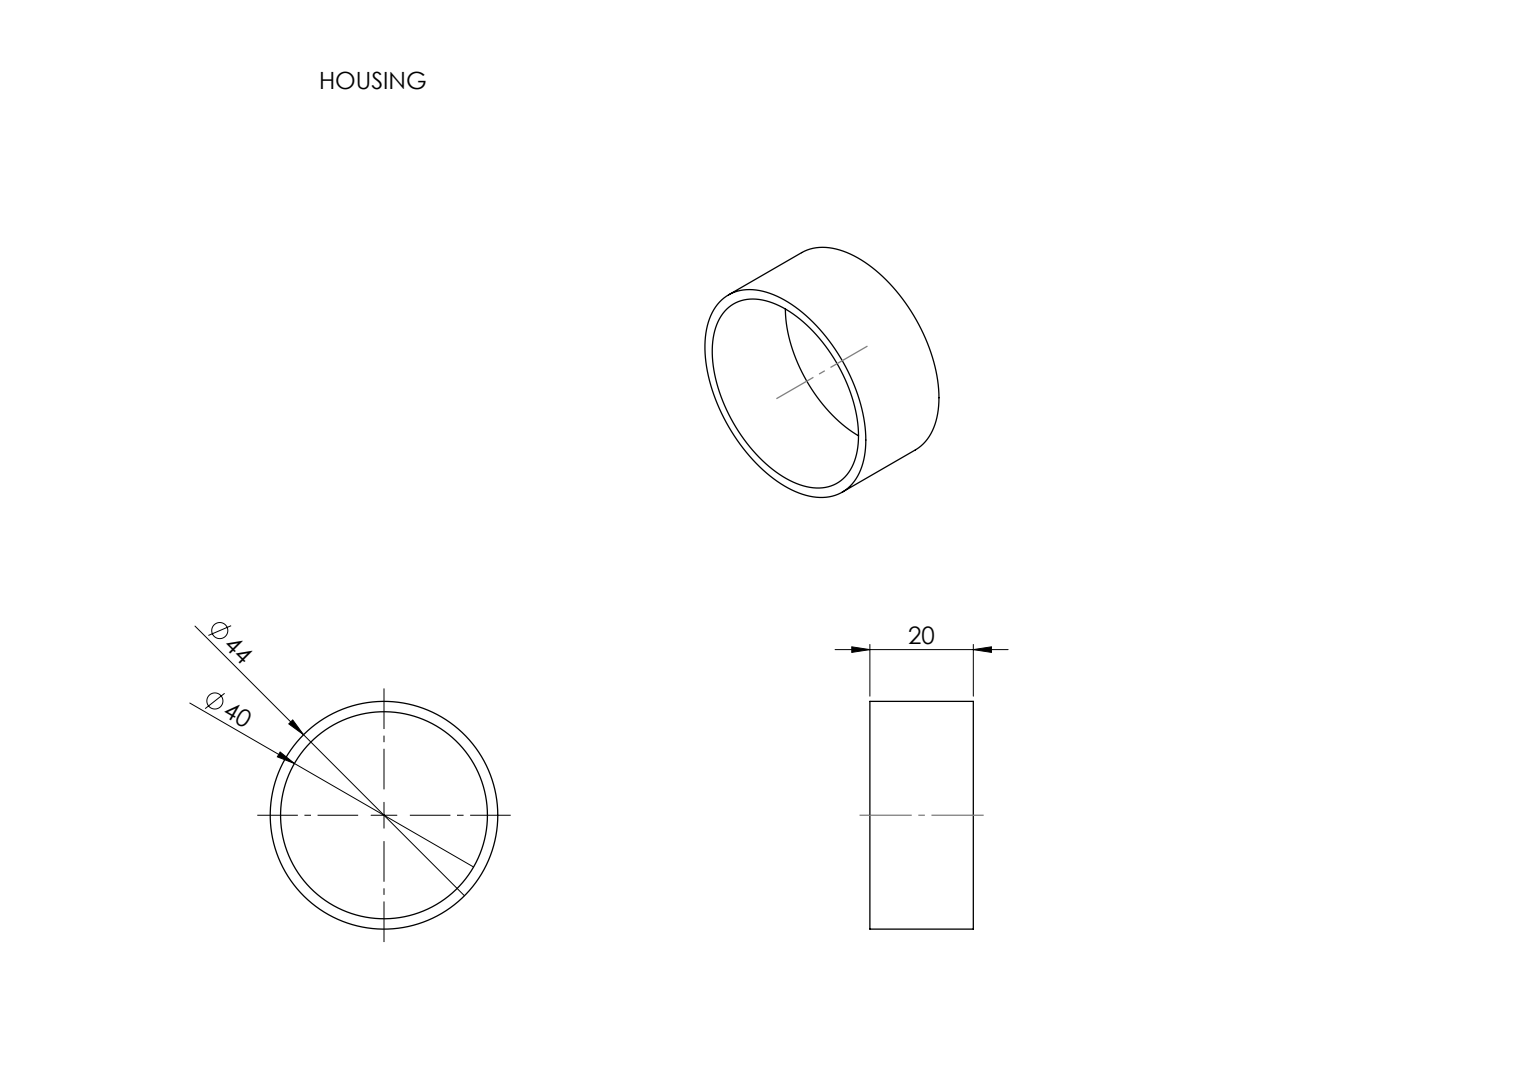
ISO-10303-21;
HEADER;
FILE_DESCRIPTION (('STEP AP214'),
    '1' );
FILE_NAME ('housing.step',
    '2026-10-08T12:30:53',
    ( '' ),
    ( '' ),
    'SwSTEP 2.0',
    'SolidWorks 2026',
    '' );
FILE_SCHEMA (( 'AUTOMOTIVE_DESIGN' ));
ENDSEC;

DATA;
#96=ORIENTED_EDGE ( 'NONE', *, *, #6796, .F. ) ;
#313=CARTESIAN_POINT ( 'NONE',  ( 0.000000000000000000, 0.000000000000000000, 20.00000000000000000 ) ) ;
#321=CARTESIAN_POINT ( 'NONE',  ( 0.000000000000000000, 0.000000000000000000, 20.00000000000000000 ) ) ;
#331=CARTESIAN_POINT ( 'NONE',  ( 0.000000000000000000, 0.000000000000000000, 20.00000000000000000 ) ) ;
#339=AXIS2_PLACEMENT_3D ( 'NONE', #331, #5047, #8783 ) ;
#478=UNCERTAINTY_MEASURE_WITH_UNIT (LENGTH_MEASURE( 1.000000000000000082E-05 ), #5286, 'distance_accuracy_value', 'NONE');
#542=DIRECTION ( 'NONE',  ( 1.000000000000000000, 0.000000000000000000, 0.000000000000000000 ) ) ;
#621=FILL_AREA_STYLE ('',( #9865 ) ) ;
#694=SURFACE_STYLE_USAGE ( .BOTH. , #4367 ) ;
#720=PRODUCT_DEFINITION_CONTEXT ( 'detailed design', #10992, 'design' ) ;
#831=CARTESIAN_POINT ( 'NONE',  ( 19.99999999999999645, 2.449293598294706119E-15, 20.00000000000000000 ) ) ;
#894=FACE_OUTER_BOUND ( 'NONE', #9272, .T. ) ;
#945=DIRECTION ( 'NONE',  ( -0.000000000000000000, -0.000000000000000000, -1.000000000000000000 ) ) ;
#949=EDGE_LOOP ( 'NONE', ( #11530, #8082, #9226, #7103 ) ) ;
#993=CIRCLE ( 'NONE', #10561, 19.99999999999999645 ) ;
#1170=VERTEX_POINT ( 'NONE', #5918 ) ;
#1179=AXIS2_PLACEMENT_3D ( 'NONE', #3701, #8417, #7546 ) ;
#1190=PLANE ( 'NONE',  #7958 ) ;
#1294=CIRCLE ( 'NONE', #7739, 19.99999999999999645 ) ;
#1477=PRESENTATION_STYLE_ASSIGNMENT (( #10268 ) ) ;
#1490=( NAMED_UNIT ( * ) SI_UNIT ( $, .STERADIAN. ) SOLID_ANGLE_UNIT ( ) );
#1492=EDGE_CURVE ( 'NONE', #10594, #10386, #9022, .T. ) ;
#1514=PRODUCT_CONTEXT ( 'NONE', #2788, 'mechanical' ) ;
#1548=MECHANICAL_DESIGN_GEOMETRIC_PRESENTATION_REPRESENTATION('',(#9368),#5064);
#1551=DIRECTION ( 'NONE',  ( 0.000000000000000000, 0.000000000000000000, 1.000000000000000000 ) ) ;
#1565=ADVANCED_FACE ( 'NONE', ( #7489 ), #10304, .F. ) ;
#1574=EDGE_CURVE ( 'NONE', #8389, #10578, #8998, .T. ) ;
#1616=AXIS2_PLACEMENT_3D ( 'NONE', #2628, #6184, #542 ) ;
#1674=CARTESIAN_POINT ( 'NONE',  ( 0.000000000000000000, 0.000000000000000000, 0.000000000000000000 ) ) ;
#1759=ADVANCED_FACE ( 'NONE', ( #5901 ), #4004, .F. ) ;
#1811=( GEOMETRIC_REPRESENTATION_CONTEXT ( 3 ) GLOBAL_UNCERTAINTY_ASSIGNED_CONTEXT ( ( #478 ) ) GLOBAL_UNIT_ASSIGNED_CONTEXT ( ( #5286, #9878, #2599 ) ) REPRESENTATION_CONTEXT ( 'NONE', 'WORKASPACE' ) );
#1812=FACE_BOUND ( 'NONE', #10883, .T. ) ;
#1825=( NAMED_UNIT ( * ) PLANE_ANGLE_UNIT ( ) SI_UNIT ( $, .RADIAN. ) );
#1826=UNCERTAINTY_MEASURE_WITH_UNIT (LENGTH_MEASURE( 1.000000000000000082E-05 ), #3721, 'distance_accuracy_value', 'NONE');
#1955=ORIENTED_EDGE ( 'NONE', *, *, #1574, .T. ) ;
#2025=EDGE_CURVE ( 'NONE', #6334, #10386, #3812, .T. ) ;
#2134=CARTESIAN_POINT ( 'NONE',  ( 0.000000000000000000, 0.000000000000000000, 20.00000000000000000 ) ) ;
#2153=DIRECTION ( 'NONE',  ( 1.000000000000000000, 0.000000000000000000, 0.000000000000000000 ) ) ;
#2166=VECTOR ( 'NONE', #10232, 1000.000000000000000 ) ;
#2182=FACE_OUTER_BOUND ( 'NONE', #5458, .T. ) ;
#2199=FACE_OUTER_BOUND ( 'NONE', #949, .T. ) ;
#2216=AXIS2_PLACEMENT_3D ( 'NONE', #2134, #10519, #10760 ) ;
#2332=VECTOR ( 'NONE', #7364, 1000.000000000000000 ) ;
#2396=EDGE_CURVE ( 'NONE', #10386, #10594, #993, .T. ) ;
#2505=CARTESIAN_POINT ( 'NONE',  ( 0.000000000000000000, 0.000000000000000000, 0.000000000000000000 ) ) ;
#2508=CARTESIAN_POINT ( 'NONE',  ( 19.99999999999999645, 2.449293598294706119E-15, 20.00000000000000000 ) ) ;
#2599=( NAMED_UNIT ( * ) SI_UNIT ( $, .STERADIAN. ) SOLID_ANGLE_UNIT ( ) );
#2628=CARTESIAN_POINT ( 'NONE',  ( 0.000000000000000000, 0.000000000000000000, 20.00000000000000000 ) ) ;
#2653=DIRECTION ( 'NONE',  ( 1.000000000000000000, 0.000000000000000000, 0.000000000000000000 ) ) ;
#2679=SURFACE_SIDE_STYLE ('',( #5212 ) ) ;
#2709=VECTOR ( 'NONE', #7824, 1000.000000000000000 ) ;
#2743=AXIS2_PLACEMENT_3D ( 'NONE', #8356, #945, #3767 ) ;
#2788=APPLICATION_CONTEXT ( 'automotive_design' ) ;
#2839=FACE_OUTER_BOUND ( 'NONE', #6431, .T. ) ;
#2852=CARTESIAN_POINT ( 'NONE',  ( 0.000000000000000000, 0.000000000000000000, 20.00000000000000000 ) ) ;
#2998=ORIENTED_EDGE ( 'NONE', *, *, #1492, .T. ) ;
#3105=ORIENTED_EDGE ( 'NONE', *, *, #8115, .F. ) ;
#3124=CIRCLE ( 'NONE', #7411, 22.00000000000000000 ) ;
#3188=COLOUR_RGB ( '', 0.72549020, 0.75294118, 0.79215686) ;
#3482=EDGE_LOOP ( 'NONE', ( #7823, #9576, #6820, #10091 ) ) ;
#3495=DIRECTION ( 'NONE',  ( 0.000000000000000000, 0.000000000000000000, 1.000000000000000000 ) ) ;
#3497=ORIENTED_EDGE ( 'NONE', *, *, #9146, .F. ) ;
#3547=CIRCLE ( 'NONE', #6281, 19.99999999999999645 ) ;
#3615=ORIENTED_EDGE ( 'NONE', *, *, #5180, .F. ) ;
#3643=CARTESIAN_POINT ( 'NONE',  ( 0.000000000000000000, 0.000000000000000000, 0.000000000000000000 ) ) ;
#3672=ORIENTED_EDGE ( 'NONE', *, *, #1574, .F. ) ;
#3692=AXIS2_PLACEMENT_3D ( 'NONE', #6399, #5550, #3710 ) ;
#3701=CARTESIAN_POINT ( 'NONE',  ( 0.000000000000000000, 0.000000000000000000, 0.000000000000000000 ) ) ;
#3710=DIRECTION ( 'NONE',  ( 1.000000000000000000, 0.000000000000000000, -0.000000000000000000 ) ) ;
#3721=( LENGTH_UNIT ( ) NAMED_UNIT ( * ) SI_UNIT ( .MILLI., .METRE. ) );
#3724=CARTESIAN_POINT ( 'NONE',  ( 19.99999999999999645, 2.449293598294706119E-15, 0.000000000000000000 ) ) ;
#3767=DIRECTION ( 'NONE',  ( -1.000000000000000000, 0.000000000000000000, 0.000000000000000000 ) ) ;
#3812=LINE ( 'NONE', #5584, #2166 ) ;
#3830=EDGE_CURVE ( 'NONE', #6334, #3911, #3547, .T. ) ;
#3872=DIRECTION ( 'NONE',  ( -1.000000000000000000, 0.000000000000000000, 0.000000000000000000 ) ) ;
#3911=VERTEX_POINT ( 'NONE', #2508 ) ;
#4004=CYLINDRICAL_SURFACE ( 'NONE', #8423, 19.99999999999999645 ) ;
#4123=DIRECTION ( 'NONE',  ( -0.000000000000000000, -0.000000000000000000, -1.000000000000000000 ) ) ;
#4260=CARTESIAN_POINT ( 'NONE',  ( -22.00000000000000000, 0.000000000000000000, 20.00000000000000000 ) ) ;
#4367=SURFACE_SIDE_STYLE ('',( #11042 ) ) ;
#4427=SHAPE_REPRESENTATION_RELATIONSHIP ( 'NONE' , 'NONE' ,  #5127, #6320 ) ;
#4454=DIRECTION ( 'NONE',  ( 0.000000000000000000, 0.000000000000000000, 1.000000000000000000 ) ) ;
#4502=AXIS2_PLACEMENT_3D ( 'NONE', #3643, #12018, #6393 ) ;
#4529=CLOSED_SHELL ( 'NONE', ( #1759, #5007, #6067, #8839, #6656, #1565 ) ) ;
#4673=CARTESIAN_POINT ( 'NONE',  ( 0.000000000000000000, 0.000000000000000000, 20.00000000000000000 ) ) ;
#4752=DIRECTION ( 'NONE',  ( 0.000000000000000000, 0.000000000000000000, 1.000000000000000000 ) ) ;
#4980=LINE ( 'NONE', #8833, #6405 ) ;
#5007=ADVANCED_FACE ( 'NONE', ( #2199 ), #11673, .T. ) ;
#5047=DIRECTION ( 'NONE',  ( 0.000000000000000000, 0.000000000000000000, 1.000000000000000000 ) ) ;
#5064=( GEOMETRIC_REPRESENTATION_CONTEXT ( 3 ) GLOBAL_UNCERTAINTY_ASSIGNED_CONTEXT ( ( #1826 ) ) GLOBAL_UNIT_ASSIGNED_CONTEXT ( ( #3721, #1825, #5499 ) ) REPRESENTATION_CONTEXT ( 'NONE', 'WORKASPACE' ) );
#5127=SHAPE_REPRESENTATION ( 'housing', ( #8474 ), #5529 ) ;
#5180=EDGE_CURVE ( 'NONE', #10578, #8389, #3124, .T. ) ;
#5205=DIRECTION ( 'NONE',  ( 1.000000000000000000, 0.000000000000000000, 0.000000000000000000 ) ) ;
#5212=SURFACE_STYLE_FILL_AREA ( #621 ) ;
#5286=( LENGTH_UNIT ( ) NAMED_UNIT ( * ) SI_UNIT ( .MILLI., .METRE. ) );
#5381=DIRECTION ( 'NONE',  ( 1.000000000000000000, 0.000000000000000000, 0.000000000000000000 ) ) ;
#5382=UNCERTAINTY_MEASURE_WITH_UNIT (LENGTH_MEASURE( 1.000000000000000082E-05 ), #10980, 'distance_accuracy_value', 'NONE');
#5458=EDGE_LOOP ( 'NONE', ( #8805, #11887 ) ) ;
#5499=( NAMED_UNIT ( * ) SI_UNIT ( $, .STERADIAN. ) SOLID_ANGLE_UNIT ( ) );
#5529=( GEOMETRIC_REPRESENTATION_CONTEXT ( 3 ) GLOBAL_UNCERTAINTY_ASSIGNED_CONTEXT ( ( #5382 ) ) GLOBAL_UNIT_ASSIGNED_CONTEXT ( ( #10980, #10861, #1490 ) ) REPRESENTATION_CONTEXT ( 'NONE', 'WORKASPACE' ) );
#5550=DIRECTION ( 'NONE',  ( 0.000000000000000000, 0.000000000000000000, 1.000000000000000000 ) ) ;
#5584=CARTESIAN_POINT ( 'NONE',  ( -19.99999999999999645, 0.000000000000000000, 20.00000000000000000 ) ) ;
#5713=ORIENTED_EDGE ( 'NONE', *, *, #9658, .T. ) ;
#5901=FACE_OUTER_BOUND ( 'NONE', #8272, .T. ) ;
#5918=CARTESIAN_POINT ( 'NONE',  ( 22.00000000000000000, 2.694222958124176809E-15, 20.00000000000000000 ) ) ;
#5967=CARTESIAN_POINT ( 'NONE',  ( -19.99999999999999645, 0.000000000000000000, 20.00000000000000000 ) ) ;
#6067=ADVANCED_FACE ( 'NONE', ( #2182, #8546 ), #1190, .T. ) ;
#6110=STYLED_ITEM ( 'NONE', ( #8104 ), #6320 ) ;
#6116=CARTESIAN_POINT ( 'NONE',  ( -22.00000000000000000, 0.000000000000000000, 0.000000000000000000 ) ) ;
#6184=DIRECTION ( 'NONE',  ( 0.000000000000000000, 0.000000000000000000, 1.000000000000000000 ) ) ;
#6205=FILL_AREA_STYLE ('',( #7350 ) ) ;
#6243=COLOUR_RGB ( '', 0.72549020, 0.75294118, 0.79215686) ;
#6245=DIRECTION ( 'NONE',  ( 0.000000000000000000, 0.000000000000000000, 1.000000000000000000 ) ) ;
#6281=AXIS2_PLACEMENT_3D ( 'NONE', #7658, #3495, #5205 ) ;
#6320=ADVANCED_BREP_SHAPE_REPRESENTATION ( '', ( #8430, #8474 ), #5529 ) ;
#6334=VERTEX_POINT ( 'NONE', #5967 ) ;
#6393=DIRECTION ( 'NONE',  ( 1.000000000000000000, 0.000000000000000000, 0.000000000000000000 ) ) ;
#6399=CARTESIAN_POINT ( 'NONE',  ( 0.000000000000000000, 0.000000000000000000, 0.000000000000000000 ) ) ;
#6405=VECTOR ( 'NONE', #11638, 1000.000000000000000 ) ;
#6412=CARTESIAN_POINT ( 'NONE',  ( 0.000000000000000000, 0.000000000000000000, 0.000000000000000000 ) ) ;
#6431=EDGE_LOOP ( 'NONE', ( #3105, #3497, #5713, #1955 ) ) ;
#6617=ORIENTED_EDGE ( 'NONE', *, *, #2025, .F. ) ;
#6656=ADVANCED_FACE ( 'NONE', ( #2839 ), #8590, .T. ) ;
#6796=EDGE_CURVE ( 'NONE', #3911, #6334, #1294, .T. ) ;
#6820=ORIENTED_EDGE ( 'NONE', *, *, #2025, .T. ) ;
#6821=ORIENTED_EDGE ( 'NONE', *, *, #3830, .F. ) ;
#6880=CIRCLE ( 'NONE', #1616, 22.00000000000000000 ) ;
#6902=CARTESIAN_POINT ( 'NONE',  ( 22.00000000000000000, 2.694222958124176809E-15, 20.00000000000000000 ) ) ;
#7103=ORIENTED_EDGE ( 'NONE', *, *, #9658, .F. ) ;
#7244=PLANE ( 'NONE',  #3692 ) ;
#7350=FILL_AREA_STYLE_COLOUR ( '', #3188 ) ;
#7364=DIRECTION ( 'NONE',  ( -0.000000000000000000, -0.000000000000000000, -1.000000000000000000 ) ) ;
#7411=AXIS2_PLACEMENT_3D ( 'NONE', #6412, #4454, #5381 ) ;
#7475=MECHANICAL_DESIGN_GEOMETRIC_PRESENTATION_REPRESENTATION('',(#6110),#1811);
#7489=FACE_OUTER_BOUND ( 'NONE', #3482, .T. ) ;
#7546=DIRECTION ( 'NONE',  ( 1.000000000000000000, 0.000000000000000000, 0.000000000000000000 ) ) ;
#7658=CARTESIAN_POINT ( 'NONE',  ( 0.000000000000000000, 0.000000000000000000, 20.00000000000000000 ) ) ;
#7687=ORIENTED_EDGE ( 'NONE', *, *, #2396, .F. ) ;
#7739=AXIS2_PLACEMENT_3D ( 'NONE', #313, #10535, #2153 ) ;
#7764=ORIENTED_EDGE ( 'NONE', *, *, #8315, .T. ) ;
#7823=ORIENTED_EDGE ( 'NONE', *, *, #8315, .F. ) ;
#7824=DIRECTION ( 'NONE',  ( -0.000000000000000000, -0.000000000000000000, -1.000000000000000000 ) ) ;
#7842=VERTEX_POINT ( 'NONE', #4260 ) ;
#7958=AXIS2_PLACEMENT_3D ( 'NONE', #2852, #4752, #11351 ) ;
#8082=ORIENTED_EDGE ( 'NONE', *, *, #8115, .T. ) ;
#8104=PRESENTATION_STYLE_ASSIGNMENT (( #694 ) ) ;
#8115=EDGE_CURVE ( 'NONE', #1170, #10578, #9666, .T. ) ;
#8272=EDGE_LOOP ( 'NONE', ( #10399, #7764, #7687, #6617 ) ) ;
#8315=EDGE_CURVE ( 'NONE', #3911, #10594, #11798, .T. ) ;
#8356=CARTESIAN_POINT ( 'NONE',  ( 0.000000000000000000, 0.000000000000000000, 20.00000000000000000 ) ) ;
#8389=VERTEX_POINT ( 'NONE', #6116 ) ;
#8417=DIRECTION ( 'NONE',  ( 0.000000000000000000, 0.000000000000000000, 1.000000000000000000 ) ) ;
#8418=ORIENTED_EDGE ( 'NONE', *, *, #2396, .T. ) ;
#8423=AXIS2_PLACEMENT_3D ( 'NONE', #321, #4123, #11590 ) ;
#8430=MANIFOLD_SOLID_BREP ( 'Extrude-Thin1', #4529 ) ;
#8474=AXIS2_PLACEMENT_3D ( 'NONE', #1674, #1551, #2653 ) ;
#8531=DIRECTION ( 'NONE',  ( -0.000000000000000000, -0.000000000000000000, -1.000000000000000000 ) ) ;
#8546=FACE_BOUND ( 'NONE', #11852, .T. ) ;
#8590=CYLINDRICAL_SURFACE ( 'NONE', #10283, 22.00000000000000000 ) ;
#8783=DIRECTION ( 'NONE',  ( 1.000000000000000000, 0.000000000000000000, 0.000000000000000000 ) ) ;
#8805=ORIENTED_EDGE ( 'NONE', *, *, #9146, .T. ) ;
#8833=CARTESIAN_POINT ( 'NONE',  ( -22.00000000000000000, 0.000000000000000000, 20.00000000000000000 ) ) ;
#8839=ADVANCED_FACE ( 'NONE', ( #894, #1812 ), #7244, .F. ) ;
#8998=CIRCLE ( 'NONE', #1179, 22.00000000000000000 ) ;
#9022=CIRCLE ( 'NONE', #4502, 19.99999999999999645 ) ;
#9106=SHAPE_DEFINITION_REPRESENTATION ( #11470, #5127 ) ;
#9146=EDGE_CURVE ( 'NONE', #7842, #1170, #10702, .T. ) ;
#9189=PRODUCT_DEFINITION_FORMATION_WITH_SPECIFIED_SOURCE ( 'ANY', '', #9411, .NOT_KNOWN. ) ;
#9226=ORIENTED_EDGE ( 'NONE', *, *, #5180, .T. ) ;
#9272=EDGE_LOOP ( 'NONE', ( #3672, #3615 ) ) ;
#9368=STYLED_ITEM ( 'NONE', ( #1477 ), #8430 ) ;
#9411=PRODUCT ( 'housing', 'housing', '', ( #1514 ) ) ;
#9576=ORIENTED_EDGE ( 'NONE', *, *, #6796, .T. ) ;
#9658=EDGE_CURVE ( 'NONE', #7842, #8389, #4980, .T. ) ;
#9666=LINE ( 'NONE', #6902, #2709 ) ;
#9865=FILL_AREA_STYLE_COLOUR ( '', #6243 ) ;
#9878=( NAMED_UNIT ( * ) PLANE_ANGLE_UNIT ( ) SI_UNIT ( $, .RADIAN. ) );
#10082=CARTESIAN_POINT ( 'NONE',  ( -19.99999999999999645, 0.000000000000000000, 0.000000000000000000 ) ) ;
#10091=ORIENTED_EDGE ( 'NONE', *, *, #1492, .F. ) ;
#10232=DIRECTION ( 'NONE',  ( -0.000000000000000000, -0.000000000000000000, -1.000000000000000000 ) ) ;
#10268=SURFACE_STYLE_USAGE ( .BOTH. , #2679 ) ;
#10283=AXIS2_PLACEMENT_3D ( 'NONE', #4673, #8531, #3872 ) ;
#10304=CYLINDRICAL_SURFACE ( 'NONE', #2743, 19.99999999999999645 ) ;
#10317=PRODUCT_DEFINITION ( 'UNKNOWN', '', #9189, #720 ) ;
#10386=VERTEX_POINT ( 'NONE', #10082 ) ;
#10399=ORIENTED_EDGE ( 'NONE', *, *, #3830, .T. ) ;
#10519=DIRECTION ( 'NONE',  ( -0.000000000000000000, -0.000000000000000000, -1.000000000000000000 ) ) ;
#10535=DIRECTION ( 'NONE',  ( 0.000000000000000000, 0.000000000000000000, 1.000000000000000000 ) ) ;
#10561=AXIS2_PLACEMENT_3D ( 'NONE', #2505, #6245, #12104 ) ;
#10578=VERTEX_POINT ( 'NONE', #11312 ) ;
#10594=VERTEX_POINT ( 'NONE', #3724 ) ;
#10702=CIRCLE ( 'NONE', #339, 22.00000000000000000 ) ;
#10760=DIRECTION ( 'NONE',  ( -1.000000000000000000, 0.000000000000000000, 0.000000000000000000 ) ) ;
#10861=( NAMED_UNIT ( * ) PLANE_ANGLE_UNIT ( ) SI_UNIT ( $, .RADIAN. ) );
#10883=EDGE_LOOP ( 'NONE', ( #8418, #2998 ) ) ;
#10980=( LENGTH_UNIT ( ) NAMED_UNIT ( * ) SI_UNIT ( .MILLI., .METRE. ) );
#10992=APPLICATION_CONTEXT ( 'automotive_design' ) ;
#11042=SURFACE_STYLE_FILL_AREA ( #6205 ) ;
#11312=CARTESIAN_POINT ( 'NONE',  ( 22.00000000000000000, 2.694222958124176809E-15, 0.000000000000000000 ) ) ;
#11351=DIRECTION ( 'NONE',  ( 1.000000000000000000, 0.000000000000000000, -0.000000000000000000 ) ) ;
#11470=PRODUCT_DEFINITION_SHAPE ( 'NONE', 'NONE',  #10317 ) ;
#11530=ORIENTED_EDGE ( 'NONE', *, *, #11840, .F. ) ;
#11590=DIRECTION ( 'NONE',  ( -1.000000000000000000, 0.000000000000000000, 0.000000000000000000 ) ) ;
#11638=DIRECTION ( 'NONE',  ( -0.000000000000000000, -0.000000000000000000, -1.000000000000000000 ) ) ;
#11673=CYLINDRICAL_SURFACE ( 'NONE', #2216, 22.00000000000000000 ) ;
#11798=LINE ( 'NONE', #831, #2332 ) ;
#11840=EDGE_CURVE ( 'NONE', #1170, #7842, #6880, .T. ) ;
#11852=EDGE_LOOP ( 'NONE', ( #6821, #96 ) ) ;
#11887=ORIENTED_EDGE ( 'NONE', *, *, #11840, .T. ) ;
#12018=DIRECTION ( 'NONE',  ( 0.000000000000000000, 0.000000000000000000, 1.000000000000000000 ) ) ;
#12104=DIRECTION ( 'NONE',  ( 1.000000000000000000, 0.000000000000000000, 0.000000000000000000 ) ) ;
ENDSEC;
END-ISO-10303-21;
